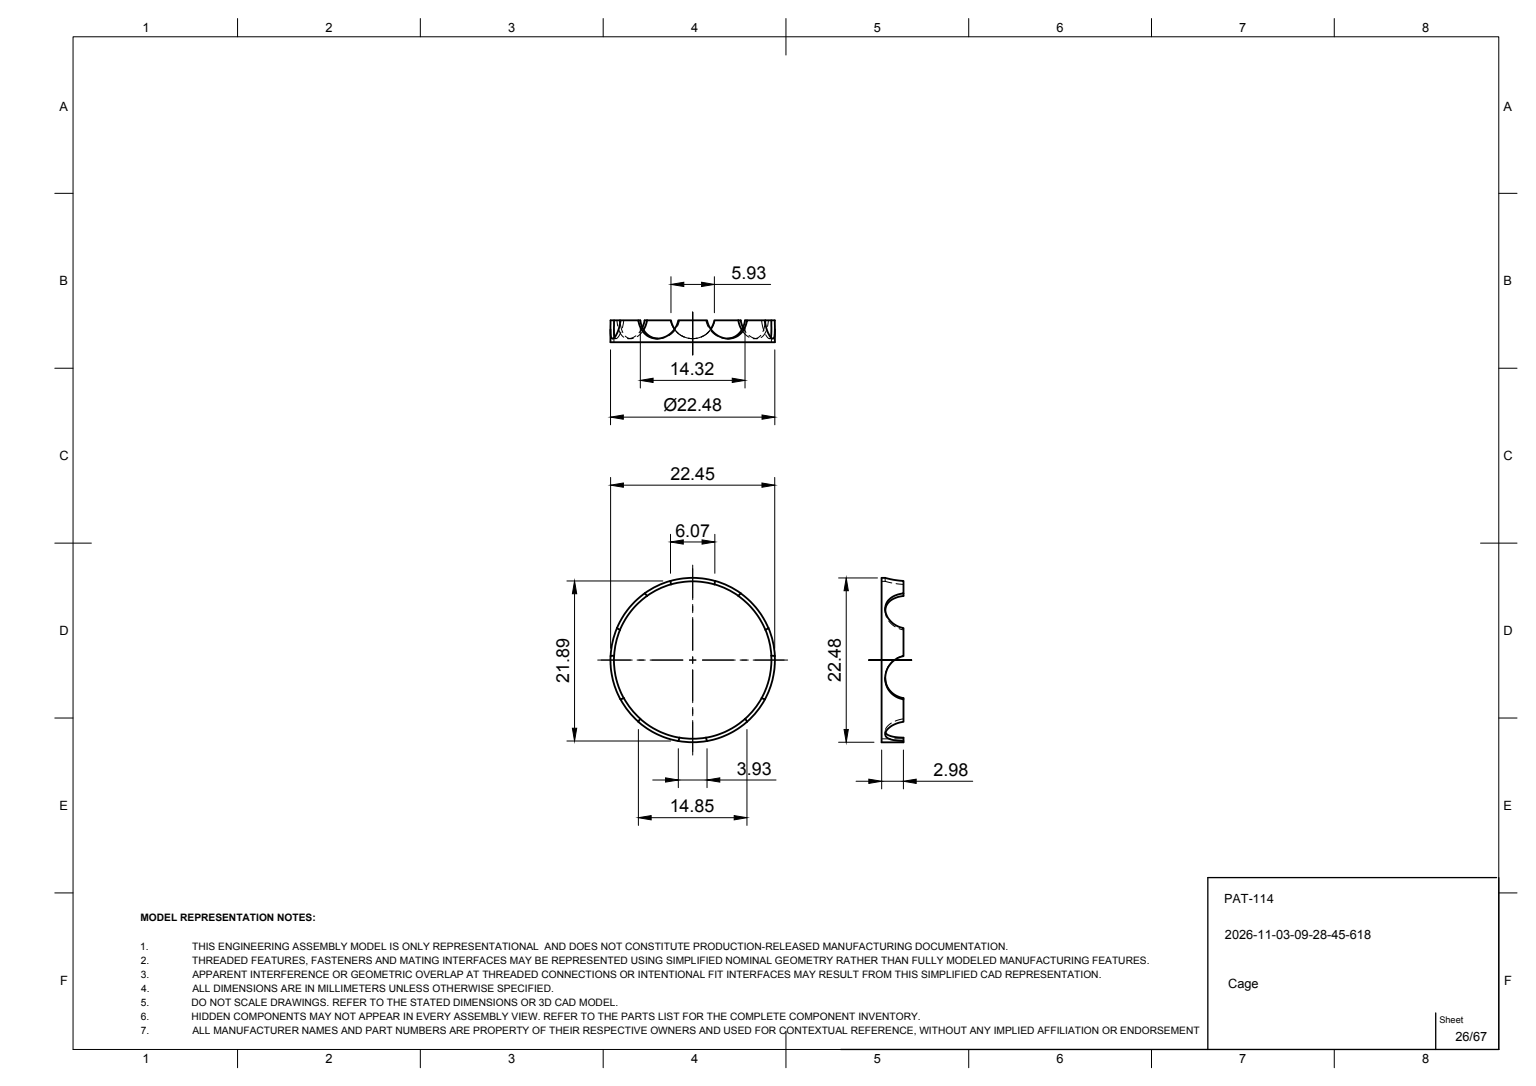
ISO-10303-21;
HEADER;
/* Generated by software containing ST-Developer
 * from STEP Tools, Inc. (www.steptools.com) 
 */

FILE_DESCRIPTION(
/* description */ ('Two-stage gear reducer in split housing'),
/* implementation_level */ '2;1');

FILE_NAME(
/* name */ 'Cage.step',
/* time_stamp */ '2026-10-28T03:22:31-07:00',
/* author */ (''),
/* organization */ (''),
/* preprocessor_version */ 'ST-DEVELOPER v20.2',
/* originating_system */ 'Autodesk Translation Framework v15.17.0.0',
/* authorisation */ '');

FILE_SCHEMA (('AUTOMOTIVE_DESIGN { 1 0 10303 214 3 1 1 }'));
ENDSEC;

DATA;
#10=MECHANICAL_DESIGN_GEOMETRIC_PRESENTATION_REPRESENTATION('',(#1260),#73366);
#931=B_SPLINE_CURVE_WITH_KNOTS('',3,(#24284,#24285,#24286,#24287,#24288,
#24289,#24290,#24291,#24292,#24293,#24294,#24295,#24296,#24297,#24298,#24299,
#24300,#24301,#24302,#24303,#24304,#24305),.UNSPECIFIED.,.F.,.F.,(4,2,2,
2,2,2,2,2,2,2,4),(0.0591825211272536,0.157966726598481,0.236950089897721,
0.315933453196962,0.391576304923761,0.46721915665056,0.54286200837736,0.618504860104159,
0.697488223403399,0.77647158670264,0.875255792173867),.UNSPECIFIED.);
#932=B_SPLINE_CURVE_WITH_KNOTS('',3,(#24309,#24310,#24311,#24312,#24313,
#24314,#24315,#24316,#24317,#24318,#24319,#24320,#24321,#24322,#24323,#24324,
#24325,#24326,#24327,#24328,#24329,#24330),.UNSPECIFIED.,.F.,.F.,(4,2,2,
2,2,2,2,2,2,2,4),(0.0581119756758434,0.106553146291161,0.213106292582322,
0.30849933801665,0.386091982889075,0.4636846277615,0.541277272633925,0.61886991750635,
0.714262962940678,0.820816109231839,0.869257279847157),.UNSPECIFIED.);
#933=B_SPLINE_CURVE_WITH_KNOTS('',3,(#24336,#24337,#24338,#24339,#24340,
#24341,#24342,#24343,#24344,#24345,#24346,#24347,#24348,#24349,#24350,#24351,
#24352,#24353,#24354,#24355,#24356,#24357),.UNSPECIFIED.,.F.,.F.,(4,2,2,
2,2,2,2,2,2,2,4),(0.0581119756758434,0.106553146291161,0.213106292582322,
0.30849933801665,0.386091982889075,0.4636846277615,0.541277272633925,0.61886991750635,
0.714262962940679,0.820816109231839,0.869257279847157),.UNSPECIFIED.);
#934=B_SPLINE_CURVE_WITH_KNOTS('',3,(#24361,#24362,#24363,#24364,#24365,
#24366,#24367,#24368,#24369,#24370,#24371,#24372,#24373,#24374,#24375,#24376,
#24377,#24378,#24379,#24380,#24381,#24382),.UNSPECIFIED.,.F.,.F.,(4,2,2,
2,2,2,2,2,2,2,4),(0.0581119756758433,0.106553146291161,0.213106292582322,
0.308499338016649,0.386091982889075,0.4636846277615,0.541277272633925,0.61886991750635,
0.714262962940678,0.820816109231839,0.869257279847157),.UNSPECIFIED.);
#935=B_SPLINE_CURVE_WITH_KNOTS('',3,(#24391,#24392,#24393,#24394,#24395,
#24396,#24397,#24398,#24399,#24400,#24401,#24402,#24403,#24404,#24405,#24406,
#24407,#24408,#24409,#24410,#24411,#24412),.UNSPECIFIED.,.F.,.F.,(4,2,2,
2,2,2,2,2,2,2,4),(0.0581119756758433,0.106553146291161,0.213106292582322,
0.30849933801665,0.386091982889075,0.4636846277615,0.541277272633925,0.61886991750635,
0.714262962940678,0.820816109231839,0.869257279847157),.UNSPECIFIED.);
#936=B_SPLINE_CURVE_WITH_KNOTS('',3,(#24416,#24417,#24418,#24419,#24420,
#24421,#24422,#24423,#24424,#24425,#24426,#24427,#24428,#24429,#24430,#24431,
#24432,#24433,#24434,#24435,#24436,#24437),.UNSPECIFIED.,.F.,.F.,(4,2,2,
2,2,2,2,2,2,2,4),(0.0581119756758434,0.106553146291161,0.213106292582322,
0.30849933801665,0.386091982889075,0.4636846277615,0.541277272633925,0.61886991750635,
0.714262962940678,0.820816109231839,0.869257279847157),.UNSPECIFIED.);
#937=B_SPLINE_CURVE_WITH_KNOTS('',3,(#24441,#24442,#24443,#24444,#24445,
#24446,#24447,#24448,#24449,#24450,#24451,#24452,#24453,#24454,#24455,#24456,
#24457,#24458,#24459,#24460,#24461,#24462),.UNSPECIFIED.,.F.,.F.,(4,2,2,
2,2,2,2,2,2,2,4),(0.0581119756758434,0.106553146291161,0.213106292582322,
0.30849933801665,0.386091982889075,0.4636846277615,0.541277272633925,0.61886991750635,
0.714262962940678,0.820816109231839,0.869257279847157),.UNSPECIFIED.);
#938=B_SPLINE_CURVE_WITH_KNOTS('',3,(#24466,#24467,#24468,#24469,#24470,
#24471,#24472,#24473,#24474,#24475,#24476,#24477,#24478,#24479,#24480,#24481,
#24482,#24483,#24484,#24485,#24486,#24487),.UNSPECIFIED.,.F.,.F.,(4,2,2,
2,2,2,2,2,2,2,4),(0.0581119756758433,0.106553146291161,0.213106292582322,
0.30849933801665,0.386091982889075,0.4636846277615,0.541277272633925,0.61886991750635,
0.714262962940678,0.820816109231839,0.869257279847157),.UNSPECIFIED.);
#939=B_SPLINE_CURVE_WITH_KNOTS('',3,(#24495,#24496,#24497,#24498,#24499,
#24500,#24501,#24502,#24503,#24504,#24505,#24506,#24507,#24508,#24509,#24510,
#24511,#24512,#24513,#24514,#24515,#24516),.UNSPECIFIED.,.F.,.F.,(4,2,2,
2,2,2,2,2,2,2,4),(0.0591825211272536,0.157966726598481,0.236950089897721,
0.315933453196962,0.391576304923761,0.467219156650561,0.54286200837736,
0.618504860104159,0.697488223403399,0.77647158670264,0.875255792173867),
 .UNSPECIFIED.);
#940=B_SPLINE_CURVE_WITH_KNOTS('',3,(#24524,#24525,#24526,#24527,#24528,
#24529,#24530,#24531,#24532,#24533,#24534,#24535,#24536,#24537,#24538,#24539,
#24540,#24541,#24542,#24543,#24544,#24545),.UNSPECIFIED.,.F.,.F.,(4,2,2,
2,2,2,2,2,2,2,4),(0.0591825211272536,0.157966726598481,0.236950089897722,
0.315933453196962,0.391576304923761,0.467219156650561,0.54286200837736,
0.618504860104159,0.697488223403399,0.77647158670264,0.875255792173867),
 .UNSPECIFIED.);
#941=B_SPLINE_CURVE_WITH_KNOTS('',3,(#24555,#24556,#24557,#24558,#24559,
#24560,#24561,#24562,#24563,#24564,#24565,#24566,#24567,#24568,#24569,#24570,
#24571,#24572,#24573,#24574,#24575,#24576),.UNSPECIFIED.,.F.,.F.,(4,2,2,
2,2,2,2,2,2,2,4),(0.0591825211272536,0.157966726598481,0.236950089897721,
0.315933453196962,0.391576304923761,0.46721915665056,0.54286200837736,0.618504860104159,
0.697488223403399,0.77647158670264,0.875255792173867),.UNSPECIFIED.);
#942=B_SPLINE_CURVE_WITH_KNOTS('',3,(#24584,#24585,#24586,#24587,#24588,
#24589,#24590,#24591,#24592,#24593,#24594,#24595,#24596,#24597,#24598,#24599,
#24600,#24601,#24602,#24603,#24604,#24605),.UNSPECIFIED.,.F.,.F.,(4,2,2,
2,2,2,2,2,2,2,4),(0.0591825211272536,0.157966726598481,0.236950089897721,
0.315933453196962,0.391576304923761,0.46721915665056,0.542862008377359,
0.618504860104159,0.697488223403399,0.776471586702639,0.875255792173867),
 .UNSPECIFIED.);
#943=B_SPLINE_CURVE_WITH_KNOTS('',3,(#24613,#24614,#24615,#24616,#24617,
#24618,#24619,#24620,#24621,#24622,#24623,#24624,#24625,#24626,#24627,#24628,
#24629,#24630,#24631,#24632,#24633,#24634),.UNSPECIFIED.,.F.,.F.,(4,2,2,
2,2,2,2,2,2,2,4),(0.0591825211272536,0.157966726598481,0.236950089897721,
0.315933453196962,0.391576304923761,0.46721915665056,0.54286200837736,0.618504860104159,
0.697488223403399,0.77647158670264,0.875255792173867),.UNSPECIFIED.);
#944=B_SPLINE_CURVE_WITH_KNOTS('',3,(#24643,#24644,#24645,#24646,#24647,
#24648,#24649,#24650,#24651,#24652,#24653,#24654,#24655,#24656,#24657,#24658,
#24659,#24660,#24661,#24662,#24663,#24664),.UNSPECIFIED.,.F.,.F.,(4,2,2,
2,2,2,2,2,2,2,4),(0.0591825211272536,0.157966726598481,0.236950089897721,
0.315933453196962,0.391576304923761,0.46721915665056,0.542862008377359,
0.618504860104159,0.697488223403399,0.776471586702639,0.875255792173867),
 .UNSPECIFIED.);
#1074=SPHERICAL_SURFACE('',#17473,0.309556);
#1075=SPHERICAL_SURFACE('',#17489,0.309556);
#1076=SPHERICAL_SURFACE('',#17494,0.309556);
#1077=SPHERICAL_SURFACE('',#17500,0.309556);
#1078=SPHERICAL_SURFACE('',#17505,0.309556);
#1079=SPHERICAL_SURFACE('',#17510,0.309556);
#1080=SPHERICAL_SURFACE('',#17518,0.309556);
#1142=SHAPE_REPRESENTATION_RELATIONSHIP('SRR','None',#73630,#1198);
#1198=ADVANCED_BREP_SHAPE_REPRESENTATION('',(#1330),#73326);
#1260=STYLED_ITEM('',(#73988),#1330);
#1330=MANIFOLD_SOLID_BREP('Continuous crown cage',#16149);
#1523=FACE_BOUND('',#3401,.T.);
#1759=PLANE('',#17486);
#1760=PLANE('',#17491);
#1761=PLANE('',#17496);
#1762=PLANE('',#17502);
#1763=PLANE('',#17507);
#1764=PLANE('',#17516);
#1765=PLANE('',#17520);
#1766=PLANE('',#17521);
#2323=FACE_OUTER_BOUND('',#3385,.T.);
#2324=FACE_OUTER_BOUND('',#3386,.T.);
#2325=FACE_OUTER_BOUND('',#3387,.T.);
#2326=FACE_OUTER_BOUND('',#3388,.T.);
#2327=FACE_OUTER_BOUND('',#3389,.T.);
#2328=FACE_OUTER_BOUND('',#3390,.T.);
#2329=FACE_OUTER_BOUND('',#3391,.T.);
#2330=FACE_OUTER_BOUND('',#3392,.T.);
#2331=FACE_OUTER_BOUND('',#3393,.T.);
#2332=FACE_OUTER_BOUND('',#3394,.T.);
#2333=FACE_OUTER_BOUND('',#3395,.T.);
#2334=FACE_OUTER_BOUND('',#3396,.T.);
#2335=FACE_OUTER_BOUND('',#3397,.T.);
#2336=FACE_OUTER_BOUND('',#3398,.T.);
#2337=FACE_OUTER_BOUND('',#3399,.T.);
#2338=FACE_OUTER_BOUND('',#3400,.T.);
#2339=FACE_OUTER_BOUND('',#3402,.T.);
#3385=EDGE_LOOP('',(#11893,#11894,#11895,#11896));
#3386=EDGE_LOOP('',(#11897,#11898,#11899,#11900,#11901,#11902,#11903,#11904,
#11905,#11906,#11907,#11908,#11909,#11910,#11911,#11912,#11913,#11914));
#3387=EDGE_LOOP('',(#11915,#11916,#11917,#11918));
#3388=EDGE_LOOP('',(#11919,#11920,#11921,#11922));
#3389=EDGE_LOOP('',(#11923,#11924,#11925,#11926));
#3390=EDGE_LOOP('',(#11927,#11928,#11929,#11930));
#3391=EDGE_LOOP('',(#11931,#11932,#11933,#11934,#11935,#11936));
#3392=EDGE_LOOP('',(#11937,#11938,#11939,#11940));
#3393=EDGE_LOOP('',(#11941,#11942,#11943,#11944));
#3394=EDGE_LOOP('',(#11945,#11946,#11947,#11948));
#3395=EDGE_LOOP('',(#11949,#11950,#11951,#11952));
#3396=EDGE_LOOP('',(#11953,#11954,#11955,#11956));
#3397=EDGE_LOOP('',(#11957,#11958,#11959,#11960,#11961,#11962,#11963,#11964,
#11965,#11966,#11967,#11968,#11969,#11970,#11971,#11972,#11973,#11974));
#3398=EDGE_LOOP('',(#11975,#11976,#11977,#11978));
#3399=EDGE_LOOP('',(#11979,#11980,#11981,#11982));
#3400=EDGE_LOOP('',(#11983));
#3401=EDGE_LOOP('',(#11984));
#3402=EDGE_LOOP('',(#11985,#11986,#11987,#11988));
#4433=LINE('',#24386,#5457);
#4434=LINE('',#24639,#5458);
#5457=VECTOR('',#20171,1.123812);
#5458=VECTOR('',#20240,1.076188);
#6420=CIRCLE('',#17474,0.303778037777585);
#6421=CIRCLE('',#17475,0.303778037777585);
#6422=CIRCLE('',#17477,1.123812);
#6423=CIRCLE('',#17478,1.123812);
#6424=CIRCLE('',#17479,1.123812);
#6425=CIRCLE('',#17480,1.123812);
#6426=CIRCLE('',#17481,1.123812);
#6427=CIRCLE('',#17482,1.123812);
#6428=CIRCLE('',#17483,1.123812);
#6429=CIRCLE('',#17484,1.123812);
#6430=CIRCLE('',#17485,1.123812);
#6431=CIRCLE('',#17487,1.076188);
#6432=CIRCLE('',#17488,0.303778037777585);
#6433=CIRCLE('',#17490,0.303778037777585);
#6434=CIRCLE('',#17492,1.076188);
#6435=CIRCLE('',#17493,0.303778037777585);
#6436=CIRCLE('',#17495,0.303778037777585);
#6437=CIRCLE('',#17497,1.076188);
#6438=CIRCLE('',#17498,1.076188);
#6439=CIRCLE('',#17499,0.303778037777585);
#6440=CIRCLE('',#17501,0.303778037777585);
#6441=CIRCLE('',#17503,1.076188);
#6442=CIRCLE('',#17504,0.303778037777585);
#6443=CIRCLE('',#17506,0.303778037777585);
#6444=CIRCLE('',#17508,1.076188);
#6445=CIRCLE('',#17509,0.303778037777585);
#6446=CIRCLE('',#17511,0.303778037777585);
#6447=CIRCLE('',#17513,1.076188);
#6448=CIRCLE('',#17514,1.076188);
#6449=CIRCLE('',#17515,1.076188);
#6450=CIRCLE('',#17517,0.303778037777585);
#6451=CIRCLE('',#17519,0.303778037777585);
#7293=VERTEX_POINT('',#24282);
#7294=VERTEX_POINT('',#24283);
#7295=VERTEX_POINT('',#24306);
#7296=VERTEX_POINT('',#24308);
#7297=VERTEX_POINT('',#24333);
#7298=VERTEX_POINT('',#24335);
#7299=VERTEX_POINT('',#24358);
#7300=VERTEX_POINT('',#24360);
#7301=VERTEX_POINT('',#24383);
#7302=VERTEX_POINT('',#24385);
#7303=VERTEX_POINT('',#24388);
#7304=VERTEX_POINT('',#24390);
#7305=VERTEX_POINT('',#24413);
#7306=VERTEX_POINT('',#24415);
#7307=VERTEX_POINT('',#24438);
#7308=VERTEX_POINT('',#24440);
#7309=VERTEX_POINT('',#24463);
#7310=VERTEX_POINT('',#24465);
#7311=VERTEX_POINT('',#24490);
#7312=VERTEX_POINT('',#24494);
#7313=VERTEX_POINT('',#24519);
#7314=VERTEX_POINT('',#24523);
#7315=VERTEX_POINT('',#24548);
#7316=VERTEX_POINT('',#24550);
#7317=VERTEX_POINT('',#24554);
#7318=VERTEX_POINT('',#24579);
#7319=VERTEX_POINT('',#24583);
#7320=VERTEX_POINT('',#24608);
#7321=VERTEX_POINT('',#24612);
#7322=VERTEX_POINT('',#24637);
#7323=VERTEX_POINT('',#24640);
#7324=VERTEX_POINT('',#24642);
#9000=EDGE_CURVE('',#7293,#7294,#931,.T.);
#9001=EDGE_CURVE('',#7295,#7293,#6420,.T.);
#9002=EDGE_CURVE('',#7296,#7295,#932,.T.);
#9003=EDGE_CURVE('',#7294,#7296,#6421,.T.);
#9004=EDGE_CURVE('',#7297,#7295,#6422,.T.);
#9005=EDGE_CURVE('',#7297,#7298,#933,.T.);
#9006=EDGE_CURVE('',#7299,#7298,#6423,.T.);
#9007=EDGE_CURVE('',#7299,#7300,#934,.T.);
#9008=EDGE_CURVE('',#7301,#7300,#6424,.T.);
#9009=EDGE_CURVE('',#7301,#7302,#4433,.T.);
#9010=EDGE_CURVE('',#7302,#7302,#6425,.T.);
#9011=EDGE_CURVE('',#7303,#7301,#6426,.T.);
#9012=EDGE_CURVE('',#7303,#7304,#935,.T.);
#9013=EDGE_CURVE('',#7305,#7304,#6427,.T.);
#9014=EDGE_CURVE('',#7305,#7306,#936,.T.);
#9015=EDGE_CURVE('',#7307,#7306,#6428,.T.);
#9016=EDGE_CURVE('',#7307,#7308,#937,.T.);
#9017=EDGE_CURVE('',#7309,#7308,#6429,.T.);
#9018=EDGE_CURVE('',#7309,#7310,#938,.T.);
#9019=EDGE_CURVE('',#7296,#7310,#6430,.T.);
#9020=EDGE_CURVE('',#7293,#7311,#6431,.T.);
#9021=EDGE_CURVE('',#7311,#7297,#6432,.T.);
#9022=EDGE_CURVE('',#7312,#7311,#939,.T.);
#9023=EDGE_CURVE('',#7298,#7312,#6433,.T.);
#9024=EDGE_CURVE('',#7312,#7313,#6434,.T.);
#9025=EDGE_CURVE('',#7313,#7299,#6435,.T.);
#9026=EDGE_CURVE('',#7314,#7313,#940,.T.);
#9027=EDGE_CURVE('',#7300,#7314,#6436,.T.);
#9028=EDGE_CURVE('',#7314,#7315,#6437,.T.);
#9029=EDGE_CURVE('',#7315,#7316,#6438,.T.);
#9030=EDGE_CURVE('',#7316,#7303,#6439,.T.);
#9031=EDGE_CURVE('',#7317,#7316,#941,.T.);
#9032=EDGE_CURVE('',#7304,#7317,#6440,.T.);
#9033=EDGE_CURVE('',#7317,#7318,#6441,.T.);
#9034=EDGE_CURVE('',#7318,#7305,#6442,.T.);
#9035=EDGE_CURVE('',#7319,#7318,#942,.T.);
#9036=EDGE_CURVE('',#7306,#7319,#6443,.T.);
#9037=EDGE_CURVE('',#7319,#7320,#6444,.T.);
#9038=EDGE_CURVE('',#7320,#7307,#6445,.T.);
#9039=EDGE_CURVE('',#7321,#7320,#943,.T.);
#9040=EDGE_CURVE('',#7308,#7321,#6446,.T.);
#9041=EDGE_CURVE('',#7322,#7322,#6447,.T.);
#9042=EDGE_CURVE('',#7322,#7315,#4434,.T.);
#9043=EDGE_CURVE('',#7323,#7294,#6448,.T.);
#9044=EDGE_CURVE('',#7323,#7324,#944,.T.);
#9045=EDGE_CURVE('',#7321,#7324,#6449,.T.);
#9046=EDGE_CURVE('',#7310,#7323,#6450,.T.);
#9047=EDGE_CURVE('',#7324,#7309,#6451,.T.);
#11893=ORIENTED_EDGE('',*,*,#9000,.F.);
#11894=ORIENTED_EDGE('',*,*,#9001,.F.);
#11895=ORIENTED_EDGE('',*,*,#9002,.F.);
#11896=ORIENTED_EDGE('',*,*,#9003,.F.);
#11897=ORIENTED_EDGE('',*,*,#9002,.T.);
#11898=ORIENTED_EDGE('',*,*,#9004,.F.);
#11899=ORIENTED_EDGE('',*,*,#9005,.T.);
#11900=ORIENTED_EDGE('',*,*,#9006,.F.);
#11901=ORIENTED_EDGE('',*,*,#9007,.T.);
#11902=ORIENTED_EDGE('',*,*,#9008,.F.);
#11903=ORIENTED_EDGE('',*,*,#9009,.T.);
#11904=ORIENTED_EDGE('',*,*,#9010,.F.);
#11905=ORIENTED_EDGE('',*,*,#9009,.F.);
#11906=ORIENTED_EDGE('',*,*,#9011,.F.);
#11907=ORIENTED_EDGE('',*,*,#9012,.T.);
#11908=ORIENTED_EDGE('',*,*,#9013,.F.);
#11909=ORIENTED_EDGE('',*,*,#9014,.T.);
#11910=ORIENTED_EDGE('',*,*,#9015,.F.);
#11911=ORIENTED_EDGE('',*,*,#9016,.T.);
#11912=ORIENTED_EDGE('',*,*,#9017,.F.);
#11913=ORIENTED_EDGE('',*,*,#9018,.T.);
#11914=ORIENTED_EDGE('',*,*,#9019,.F.);
#11915=ORIENTED_EDGE('',*,*,#9001,.T.);
#11916=ORIENTED_EDGE('',*,*,#9020,.T.);
#11917=ORIENTED_EDGE('',*,*,#9021,.T.);
#11918=ORIENTED_EDGE('',*,*,#9004,.T.);
#11919=ORIENTED_EDGE('',*,*,#9022,.F.);
#11920=ORIENTED_EDGE('',*,*,#9023,.F.);
#11921=ORIENTED_EDGE('',*,*,#9005,.F.);
#11922=ORIENTED_EDGE('',*,*,#9021,.F.);
#11923=ORIENTED_EDGE('',*,*,#9023,.T.);
#11924=ORIENTED_EDGE('',*,*,#9024,.T.);
#11925=ORIENTED_EDGE('',*,*,#9025,.T.);
#11926=ORIENTED_EDGE('',*,*,#9006,.T.);
#11927=ORIENTED_EDGE('',*,*,#9026,.F.);
#11928=ORIENTED_EDGE('',*,*,#9027,.F.);
#11929=ORIENTED_EDGE('',*,*,#9007,.F.);
#11930=ORIENTED_EDGE('',*,*,#9025,.F.);
#11931=ORIENTED_EDGE('',*,*,#9027,.T.);
#11932=ORIENTED_EDGE('',*,*,#9028,.T.);
#11933=ORIENTED_EDGE('',*,*,#9029,.T.);
#11934=ORIENTED_EDGE('',*,*,#9030,.T.);
#11935=ORIENTED_EDGE('',*,*,#9011,.T.);
#11936=ORIENTED_EDGE('',*,*,#9008,.T.);
#11937=ORIENTED_EDGE('',*,*,#9031,.F.);
#11938=ORIENTED_EDGE('',*,*,#9032,.F.);
#11939=ORIENTED_EDGE('',*,*,#9012,.F.);
#11940=ORIENTED_EDGE('',*,*,#9030,.F.);
#11941=ORIENTED_EDGE('',*,*,#9032,.T.);
#11942=ORIENTED_EDGE('',*,*,#9033,.T.);
#11943=ORIENTED_EDGE('',*,*,#9034,.T.);
#11944=ORIENTED_EDGE('',*,*,#9013,.T.);
#11945=ORIENTED_EDGE('',*,*,#9035,.F.);
#11946=ORIENTED_EDGE('',*,*,#9036,.F.);
#11947=ORIENTED_EDGE('',*,*,#9014,.F.);
#11948=ORIENTED_EDGE('',*,*,#9034,.F.);
#11949=ORIENTED_EDGE('',*,*,#9036,.T.);
#11950=ORIENTED_EDGE('',*,*,#9037,.T.);
#11951=ORIENTED_EDGE('',*,*,#9038,.T.);
#11952=ORIENTED_EDGE('',*,*,#9015,.T.);
#11953=ORIENTED_EDGE('',*,*,#9016,.F.);
#11954=ORIENTED_EDGE('',*,*,#9038,.F.);
#11955=ORIENTED_EDGE('',*,*,#9039,.F.);
#11956=ORIENTED_EDGE('',*,*,#9040,.F.);
#11957=ORIENTED_EDGE('',*,*,#9041,.F.);
#11958=ORIENTED_EDGE('',*,*,#9042,.T.);
#11959=ORIENTED_EDGE('',*,*,#9028,.F.);
#11960=ORIENTED_EDGE('',*,*,#9026,.T.);
#11961=ORIENTED_EDGE('',*,*,#9024,.F.);
#11962=ORIENTED_EDGE('',*,*,#9022,.T.);
#11963=ORIENTED_EDGE('',*,*,#9020,.F.);
#11964=ORIENTED_EDGE('',*,*,#9000,.T.);
#11965=ORIENTED_EDGE('',*,*,#9043,.F.);
#11966=ORIENTED_EDGE('',*,*,#9044,.T.);
#11967=ORIENTED_EDGE('',*,*,#9045,.F.);
#11968=ORIENTED_EDGE('',*,*,#9039,.T.);
#11969=ORIENTED_EDGE('',*,*,#9037,.F.);
#11970=ORIENTED_EDGE('',*,*,#9035,.T.);
#11971=ORIENTED_EDGE('',*,*,#9033,.F.);
#11972=ORIENTED_EDGE('',*,*,#9031,.T.);
#11973=ORIENTED_EDGE('',*,*,#9029,.F.);
#11974=ORIENTED_EDGE('',*,*,#9042,.F.);
#11975=ORIENTED_EDGE('',*,*,#9003,.T.);
#11976=ORIENTED_EDGE('',*,*,#9019,.T.);
#11977=ORIENTED_EDGE('',*,*,#9046,.T.);
#11978=ORIENTED_EDGE('',*,*,#9043,.T.);
#11979=ORIENTED_EDGE('',*,*,#9018,.F.);
#11980=ORIENTED_EDGE('',*,*,#9047,.F.);
#11981=ORIENTED_EDGE('',*,*,#9044,.F.);
#11982=ORIENTED_EDGE('',*,*,#9046,.F.);
#11983=ORIENTED_EDGE('',*,*,#9010,.T.);
#11984=ORIENTED_EDGE('',*,*,#9041,.T.);
#11985=ORIENTED_EDGE('',*,*,#9040,.T.);
#11986=ORIENTED_EDGE('',*,*,#9045,.T.);
#11987=ORIENTED_EDGE('',*,*,#9047,.T.);
#11988=ORIENTED_EDGE('',*,*,#9017,.T.);
#15055=CYLINDRICAL_SURFACE('',#17476,1.123812);
#15056=CYLINDRICAL_SURFACE('',#17512,1.076188);
#15530=ADVANCED_FACE('',(#2323),#1074,.F.);
#15531=ADVANCED_FACE('',(#2324),#15055,.T.);
#15532=ADVANCED_FACE('',(#2325),#1759,.T.);
#15533=ADVANCED_FACE('',(#2326),#1075,.F.);
#15534=ADVANCED_FACE('',(#2327),#1760,.T.);
#15535=ADVANCED_FACE('',(#2328),#1076,.F.);
#15536=ADVANCED_FACE('',(#2329),#1761,.T.);
#15537=ADVANCED_FACE('',(#2330),#1077,.F.);
#15538=ADVANCED_FACE('',(#2331),#1762,.T.);
#15539=ADVANCED_FACE('',(#2332),#1078,.F.);
#15540=ADVANCED_FACE('',(#2333),#1763,.T.);
#15541=ADVANCED_FACE('',(#2334),#1079,.F.);
#15542=ADVANCED_FACE('',(#2335),#15056,.F.);
#15543=ADVANCED_FACE('',(#2336),#1764,.T.);
#15544=ADVANCED_FACE('',(#2337),#1080,.F.);
#15545=ADVANCED_FACE('',(#2338,#1523),#1765,.T.);
#15546=ADVANCED_FACE('',(#2339),#1766,.T.);
#16149=CLOSED_SHELL('',(#15530,#15531,#15532,#15533,#15534,#15535,#15536,
#15537,#15538,#15539,#15540,#15541,#15542,#15543,#15544,#15545,#15546));
#17472=AXIS2_PLACEMENT_3D('',#24280,#20155,#20156);
#17473=AXIS2_PLACEMENT_3D('',#24281,#20157,#20158);
#17474=AXIS2_PLACEMENT_3D('',#24307,#20159,#20160);
#17475=AXIS2_PLACEMENT_3D('',#24331,#20161,#20162);
#17476=AXIS2_PLACEMENT_3D('',#24332,#20163,#20164);
#17477=AXIS2_PLACEMENT_3D('',#24334,#20165,#20166);
#17478=AXIS2_PLACEMENT_3D('',#24359,#20167,#20168);
#17479=AXIS2_PLACEMENT_3D('',#24384,#20169,#20170);
#17480=AXIS2_PLACEMENT_3D('',#24387,#20172,#20173);
#17481=AXIS2_PLACEMENT_3D('',#24389,#20174,#20175);
#17482=AXIS2_PLACEMENT_3D('',#24414,#20176,#20177);
#17483=AXIS2_PLACEMENT_3D('',#24439,#20178,#20179);
#17484=AXIS2_PLACEMENT_3D('',#24464,#20180,#20181);
#17485=AXIS2_PLACEMENT_3D('',#24488,#20182,#20183);
#17486=AXIS2_PLACEMENT_3D('',#24489,#20184,#20185);
#17487=AXIS2_PLACEMENT_3D('',#24491,#20186,#20187);
#17488=AXIS2_PLACEMENT_3D('',#24492,#20188,#20189);
#17489=AXIS2_PLACEMENT_3D('',#24493,#20190,#20191);
#17490=AXIS2_PLACEMENT_3D('',#24517,#20192,#20193);
#17491=AXIS2_PLACEMENT_3D('',#24518,#20194,#20195);
#17492=AXIS2_PLACEMENT_3D('',#24520,#20196,#20197);
#17493=AXIS2_PLACEMENT_3D('',#24521,#20198,#20199);
#17494=AXIS2_PLACEMENT_3D('',#24522,#20200,#20201);
#17495=AXIS2_PLACEMENT_3D('',#24546,#20202,#20203);
#17496=AXIS2_PLACEMENT_3D('',#24547,#20204,#20205);
#17497=AXIS2_PLACEMENT_3D('',#24549,#20206,#20207);
#17498=AXIS2_PLACEMENT_3D('',#24551,#20208,#20209);
#17499=AXIS2_PLACEMENT_3D('',#24552,#20210,#20211);
#17500=AXIS2_PLACEMENT_3D('',#24553,#20212,#20213);
#17501=AXIS2_PLACEMENT_3D('',#24577,#20214,#20215);
#17502=AXIS2_PLACEMENT_3D('',#24578,#20216,#20217);
#17503=AXIS2_PLACEMENT_3D('',#24580,#20218,#20219);
#17504=AXIS2_PLACEMENT_3D('',#24581,#20220,#20221);
#17505=AXIS2_PLACEMENT_3D('',#24582,#20222,#20223);
#17506=AXIS2_PLACEMENT_3D('',#24606,#20224,#20225);
#17507=AXIS2_PLACEMENT_3D('',#24607,#20226,#20227);
#17508=AXIS2_PLACEMENT_3D('',#24609,#20228,#20229);
#17509=AXIS2_PLACEMENT_3D('',#24610,#20230,#20231);
#17510=AXIS2_PLACEMENT_3D('',#24611,#20232,#20233);
#17511=AXIS2_PLACEMENT_3D('',#24635,#20234,#20235);
#17512=AXIS2_PLACEMENT_3D('',#24636,#20236,#20237);
#17513=AXIS2_PLACEMENT_3D('',#24638,#20238,#20239);
#17514=AXIS2_PLACEMENT_3D('',#24641,#20241,#20242);
#17515=AXIS2_PLACEMENT_3D('',#24665,#20243,#20244);
#17516=AXIS2_PLACEMENT_3D('',#24666,#20245,#20246);
#17517=AXIS2_PLACEMENT_3D('',#24667,#20247,#20248);
#17518=AXIS2_PLACEMENT_3D('',#24668,#20249,#20250);
#17519=AXIS2_PLACEMENT_3D('',#24669,#20251,#20252);
#17520=AXIS2_PLACEMENT_3D('',#24670,#20253,#20254);
#17521=AXIS2_PLACEMENT_3D('',#24671,#20255,#20256);
#20155=DIRECTION('axis',(0.,0.,1.));
#20156=DIRECTION('refdir',(1.,0.,0.));
#20157=DIRECTION('center_axis',(0.,0.,1.));
#20158=DIRECTION('ref_axis',(1.,0.,0.));
#20159=DIRECTION('center_axis',(0.,-1.,0.));
#20160=DIRECTION('ref_axis',(0.,0.,-1.));
#20161=DIRECTION('center_axis',(0.,-1.,0.));
#20162=DIRECTION('ref_axis',(0.,0.,-1.));
#20163=DIRECTION('center_axis',(0.,1.,0.));
#20164=DIRECTION('ref_axis',(1.,0.,0.));
#20165=DIRECTION('center_axis',(0.,1.,0.));
#20166=DIRECTION('ref_axis',(1.,0.,0.));
#20167=DIRECTION('center_axis',(0.,1.,0.));
#20168=DIRECTION('ref_axis',(1.,0.,0.));
#20169=DIRECTION('center_axis',(0.,1.,0.));
#20170=DIRECTION('ref_axis',(1.,0.,0.));
#20171=DIRECTION('',(0.,-1.,0.));
#20172=DIRECTION('center_axis',(0.,-1.,0.));
#20173=DIRECTION('ref_axis',(1.,0.,0.));
#20174=DIRECTION('center_axis',(0.,1.,0.));
#20175=DIRECTION('ref_axis',(1.,0.,0.));
#20176=DIRECTION('center_axis',(0.,1.,0.));
#20177=DIRECTION('ref_axis',(1.,0.,0.));
#20178=DIRECTION('center_axis',(0.,1.,0.));
#20179=DIRECTION('ref_axis',(1.,0.,0.));
#20180=DIRECTION('center_axis',(0.,1.,0.));
#20181=DIRECTION('ref_axis',(1.,0.,0.));
#20182=DIRECTION('center_axis',(0.,1.,0.));
#20183=DIRECTION('ref_axis',(1.,0.,0.));
#20184=DIRECTION('center_axis',(0.,1.,0.));
#20185=DIRECTION('ref_axis',(1.,0.,0.));
#20186=DIRECTION('center_axis',(0.,-1.,0.));
#20187=DIRECTION('ref_axis',(1.,0.,0.));
#20188=DIRECTION('center_axis',(0.,-1.,0.));
#20189=DIRECTION('ref_axis',(0.,0.,-1.));
#20190=DIRECTION('center_axis',(8.96625347776458E-17,0.,1.));
#20191=DIRECTION('ref_axis',(1.,0.,0.));
#20192=DIRECTION('center_axis',(0.,-1.,0.));
#20193=DIRECTION('ref_axis',(0.,0.,-1.));
#20194=DIRECTION('center_axis',(0.,1.,0.));
#20195=DIRECTION('ref_axis',(1.,0.,0.));
#20196=DIRECTION('center_axis',(0.,-1.,0.));
#20197=DIRECTION('ref_axis',(1.,0.,0.));
#20198=DIRECTION('center_axis',(0.,-1.,0.));
#20199=DIRECTION('ref_axis',(0.,0.,-1.));
#20200=DIRECTION('center_axis',(0.,0.,1.));
#20201=DIRECTION('ref_axis',(1.,0.,0.));
#20202=DIRECTION('center_axis',(0.,-1.,0.));
#20203=DIRECTION('ref_axis',(0.,0.,-1.));
#20204=DIRECTION('center_axis',(0.,1.,0.));
#20205=DIRECTION('ref_axis',(1.,0.,0.));
#20206=DIRECTION('center_axis',(0.,-1.,0.));
#20207=DIRECTION('ref_axis',(1.,0.,0.));
#20208=DIRECTION('center_axis',(0.,-1.,0.));
#20209=DIRECTION('ref_axis',(1.,0.,0.));
#20210=DIRECTION('center_axis',(0.,-1.,0.));
#20211=DIRECTION('ref_axis',(0.,0.,-1.));
#20212=DIRECTION('center_axis',(0.,0.,1.));
#20213=DIRECTION('ref_axis',(1.,0.,0.));
#20214=DIRECTION('center_axis',(0.,-1.,0.));
#20215=DIRECTION('ref_axis',(0.,0.,-1.));
#20216=DIRECTION('center_axis',(0.,1.,0.));
#20217=DIRECTION('ref_axis',(1.,0.,0.));
#20218=DIRECTION('center_axis',(0.,-1.,0.));
#20219=DIRECTION('ref_axis',(1.,0.,0.));
#20220=DIRECTION('center_axis',(0.,-1.,0.));
#20221=DIRECTION('ref_axis',(0.,0.,-1.));
#20222=DIRECTION('center_axis',(8.96625347776458E-17,0.,1.));
#20223=DIRECTION('ref_axis',(1.,0.,0.));
#20224=DIRECTION('center_axis',(0.,-1.,0.));
#20225=DIRECTION('ref_axis',(0.,0.,-1.));
#20226=DIRECTION('center_axis',(0.,1.,0.));
#20227=DIRECTION('ref_axis',(1.,0.,0.));
#20228=DIRECTION('center_axis',(0.,-1.,0.));
#20229=DIRECTION('ref_axis',(1.,0.,0.));
#20230=DIRECTION('center_axis',(0.,-1.,0.));
#20231=DIRECTION('ref_axis',(0.,0.,-1.));
#20232=DIRECTION('center_axis',(0.,0.,1.));
#20233=DIRECTION('ref_axis',(1.,0.,0.));
#20234=DIRECTION('center_axis',(0.,-1.,0.));
#20235=DIRECTION('ref_axis',(0.,0.,-1.));
#20236=DIRECTION('center_axis',(0.,1.,0.));
#20237=DIRECTION('ref_axis',(1.,0.,0.));
#20238=DIRECTION('center_axis',(0.,1.,0.));
#20239=DIRECTION('ref_axis',(1.,0.,0.));
#20240=DIRECTION('',(0.,1.,0.));
#20241=DIRECTION('center_axis',(0.,-1.,0.));
#20242=DIRECTION('ref_axis',(1.,0.,0.));
#20243=DIRECTION('center_axis',(0.,-1.,0.));
#20244=DIRECTION('ref_axis',(1.,0.,0.));
#20245=DIRECTION('center_axis',(0.,1.,0.));
#20246=DIRECTION('ref_axis',(1.,0.,0.));
#20247=DIRECTION('center_axis',(0.,-1.,0.));
#20248=DIRECTION('ref_axis',(0.,0.,-1.));
#20249=DIRECTION('center_axis',(0.,0.,1.));
#20250=DIRECTION('ref_axis',(1.,0.,0.));
#20251=DIRECTION('center_axis',(0.,-1.,0.));
#20252=DIRECTION('ref_axis',(0.,0.,-1.));
#20253=DIRECTION('center_axis',(0.,-1.,0.));
#20254=DIRECTION('ref_axis',(-1.,0.,0.));
#20255=DIRECTION('center_axis',(0.,1.,0.));
#20256=DIRECTION('ref_axis',(1.,0.,0.));
#24280=CARTESIAN_POINT('',(0.,0.,0.));
#24281=CARTESIAN_POINT('Origin',(0.685838782044607,0.,0.860014630714833));
#24282=CARTESIAN_POINT('',(0.413083465285518,-0.05953,0.993751811093549));
#24283=CARTESIAN_POINT('',(0.876916659919095,-0.05953,0.623857181492959));
#24284=CARTESIAN_POINT('Ctrl Pts',(0.413083465285518,-0.05953,0.993751811093549));
#24285=CARTESIAN_POINT('Ctrl Pts',(0.419070565453383,-0.0925528133349865,
0.991263089003441));
#24286=CARTESIAN_POINT('Ctrl Pts',(0.430199341854858,-0.124911173756694,
0.986608710139579));
#24287=CARTESIAN_POINT('Ctrl Pts',(0.457978755888596,-0.177924977804098,
0.973971221090534));
#24288=CARTESIAN_POINT('Ctrl Pts',(0.473077587363685,-0.199697230012983,
0.966820759530997));
#24289=CARTESIAN_POINT('Ctrl Pts',(0.507057380724533,-0.237895043532788,
0.949440676105255));
#24290=CARTESIAN_POINT('Ctrl Pts',(0.525933334162555,-0.254319232363049,
0.939198248544428));
#24291=CARTESIAN_POINT('Ctrl Pts',(0.564362943424238,-0.28018331644634,
0.916597376014514));
#24292=CARTESIAN_POINT('Ctrl Pts',(0.585840553788742,-0.29104845371857,
0.903141581680914));
#24293=CARTESIAN_POINT('Ctrl Pts',(0.629305439856167,-0.30527573347708,
0.873412008702649));
#24294=CARTESIAN_POINT('Ctrl Pts',(0.651278921914856,-0.308638795020976,
0.857118508332695));
#24295=CARTESIAN_POINT('Ctrl Pts',(0.690705563850638,-0.308638795020976,
0.825676810575914));
#24296=CARTESIAN_POINT('Ctrl Pts',(0.711480111898423,-0.30527573347708,
0.807879894508811));
#24297=CARTESIAN_POINT('Ctrl Pts',(0.750136149454208,-0.29104845371857,
0.772120216227122));
#24298=CARTESIAN_POINT('Ctrl Pts',(0.768033796848072,-0.28018331644634,
0.754175290318038));
#24299=CARTESIAN_POINT('Ctrl Pts',(0.798619410861634,-0.254319232363049,
0.721738358858166));
#24300=CARTESIAN_POINT('Ctrl Pts',(0.812805334167529,-0.237895043532788,
0.705614819529209));
#24301=CARTESIAN_POINT('Ctrl Pts',(0.837310877969633,-0.199697230012983,
0.676354402927683));
#24302=CARTESIAN_POINT('Ctrl Pts',(0.847641868610495,-0.177924977804098,
0.663225258065736));
#24303=CARTESIAN_POINT('Ctrl Pts',(0.866144010579847,-0.124911173756694,
0.638954437806245));
#24304=CARTESIAN_POINT('Ctrl Pts',(0.873158080166742,-0.0925528133349865,
0.62914037979579));
#24305=CARTESIAN_POINT('Ctrl Pts',(0.876916659919095,-0.05953,0.623857181492959));
#24306=CARTESIAN_POINT('',(0.437601487681057,-0.05953,1.03511272300331));
#24307=CARTESIAN_POINT('Origin',(0.685838782044607,-0.05953,0.860014630714833));
#24308=CARTESIAN_POINT('',(0.911784794170997,-0.05953,0.656964154625313));
#24309=CARTESIAN_POINT('Ctrl Pts',(0.911784794170998,-0.0595300000000001,
0.656964154625312));
#24310=CARTESIAN_POINT('Ctrl Pts',(0.909827729890942,-0.0762225747374255,
0.659680317203144));
#24311=CARTESIAN_POINT('Ctrl Pts',(0.907004864562642,-0.0928409665394228,
0.663576540841106));
#24312=CARTESIAN_POINT('Ctrl Pts',(0.895234408667242,-0.144299303100741,
0.679480524217551));
#24313=CARTESIAN_POINT('Ctrl Pts',(0.882797231409153,-0.177024326825049,
0.695831250979106));
#24314=CARTESIAN_POINT('Ctrl Pts',(0.854332839576145,-0.227269801620064,
0.73042219438957));
#24315=CARTESIAN_POINT('Ctrl Pts',(0.834863020612702,-0.251265615809407,
0.752807465209441));
#24316=CARTESIAN_POINT('Ctrl Pts',(0.800439809856111,-0.279889827963178,
0.789147407129766));
#24317=CARTESIAN_POINT('Ctrl Pts',(0.781998747691871,-0.290879136862659,
0.80756613568454));
#24318=CARTESIAN_POINT('Ctrl Pts',(0.742239891936898,-0.305251990234487,
0.844254137480382));
#24319=CARTESIAN_POINT('Ctrl Pts',(0.720906778729541,-0.308638795020976,
0.862505527716294));
#24320=CARTESIAN_POINT('Ctrl Pts',(0.680463863683392,-0.308638795020976,
0.894757676234429));
#24321=CARTESIAN_POINT('Ctrl Pts',(0.657923009631182,-0.305251990234488,
0.91149460735272));
#24322=CARTESIAN_POINT('Ctrl Pts',(0.613307674922609,-0.290879136862659,
0.942092777160053));
#24323=CARTESIAN_POINT('Ctrl Pts',(0.591247219971725,-0.279889827963178,
0.955972930713954));
#24324=CARTESIAN_POINT('Ctrl Pts',(0.548158511259202,-0.251265615809407,
0.981446681891443));
#24325=CARTESIAN_POINT('Ctrl Pts',(0.522002043615455,-0.227269801620063,
0.995447160474328));
#24326=CARTESIAN_POINT('Ctrl Pts',(0.481944444320713,-0.177024326825049,
1.01550068154148));
#24327=CARTESIAN_POINT('Ctrl Pts',(0.463236132117164,-0.14429930310074,
1.0239876538093));
#24328=CARTESIAN_POINT('Ctrl Pts',(0.445111721969657,-0.0928409665394226,
1.03192403056628));
#24329=CARTESIAN_POINT('Ctrl Pts',(0.440685038163619,-0.0762225747374254,
1.03380912944435));
#24330=CARTESIAN_POINT('Ctrl Pts',(0.437601487681056,-0.05953,1.03511272300331));
#24331=CARTESIAN_POINT('Origin',(0.685838782044607,-0.05953,0.860014630714833));
#24332=CARTESIAN_POINT('Origin',(0.,-0.208355,0.));
#24333=CARTESIAN_POINT('',(0.0548532617164168,-0.05953,1.12247250791415));
#24334=CARTESIAN_POINT('Origin',(0.,-0.05953,0.));
#24335=CARTESIAN_POINT('',(-0.536443649899848,-0.05953,0.987512846410683));
#24336=CARTESIAN_POINT('Ctrl Pts',(0.0548532617164173,-0.0595300000000001,
1.12247250791414));
#24337=CARTESIAN_POINT('Ctrl Pts',(0.05150947068137,-0.0762225747374254,
1.12263591311425));
#24338=CARTESIAN_POINT('Ctrl Pts',(0.0467032526342597,-0.0928409665394227,
1.12285816383385));
#24339=CARTESIAN_POINT('Ctrl Pts',(0.0269302585198975,-0.144299303100741,
1.12357162229597));
#24340=CARTESIAN_POINT('Ctrl Pts',(0.006392292392153,-0.177024326825049,
1.12404235695137));
#24341=CARTESIAN_POINT('Ctrl Pts',(-0.0383992541984087,-0.227269801620063,
1.12335509974011));
#24342=CARTESIAN_POINT('Ctrl Pts',(-0.0680399972366993,-0.251265615809407,
1.12208997038458));
#24343=CARTESIAN_POINT('Ctrl Pts',(-0.117914228755037,-0.279889827963178,
1.1178344036749));
#24344=CARTESIAN_POINT('Ctrl Pts',(-0.14381238480104,-0.290879136862659,
1.11490049012186));
#24345=CARTESIAN_POINT('Ctrl Pts',(-0.19728546073067,-0.305251990234488,
1.10669035995599));
#24346=CARTESIAN_POINT('Ctrl Pts',(-0.224855950742601,-0.308638795020976,
1.10139101611326));
#24347=CARTESIAN_POINT('Ctrl Pts',(-0.275287440920027,-0.308638795020976,
1.0898803575765));
#24348=CARTESIAN_POINT('Ctrl Pts',(-0.302426893214945,-0.305251990234488,
1.08269251410343));
#24349=CARTESIAN_POINT('Ctrl Pts',(-0.35416671187353,-0.290879136862659,
1.06688848765783));
#24350=CARTESIAN_POINT('Ctrl Pts',(-0.3787731215897,-0.279889827963178,
1.05829506364875));
#24351=CARTESIAN_POINT('Ctrl Pts',(-0.425554672694338,-0.251265615809407,
1.04048957871266));
#24352=CARTESIAN_POINT('Ctrl Pts',(-0.452808978448581,-0.227269801620063,
1.02876878445619));
#24353=CARTESIAN_POINT('Ctrl Pts',(-0.493462957200432,-0.177024326825049,
1.0099536580922));
#24354=CARTESIAN_POINT('Ctrl Pts',(-0.511762781179148,-0.14429930310074,
1.00061845128527));
#24355=CARTESIAN_POINT('Ctrl Pts',(-0.529268075276157,-0.0928409665394226,
0.991396466802468));
#24356=CARTESIAN_POINT('Ctrl Pts',(-0.533501897135713,-0.0762225747374254,
0.989110885965947));
#24357=CARTESIAN_POINT('Ctrl Pts',(-0.536443649899848,-0.0595300000000001,
0.987512846410683));
#24358=CARTESIAN_POINT('',(-0.843383895613249,-0.05953,0.742736168477219));
#24359=CARTESIAN_POINT('Origin',(0.,-0.05953,0.));
#24360=CARTESIAN_POINT('',(-1.10653577764992,-0.05953,0.196295654879792));
#24361=CARTESIAN_POINT('Ctrl Pts',(-0.843383895613249,-0.0595300000000001,
0.742736168477219));
#24362=CARTESIAN_POINT('Ctrl Pts',(-0.84559647055299,-0.0762225747374255,
0.740223768851062));
#24363=CARTESIAN_POINT('Ctrl Pts',(-0.848766861100456,-0.0928409665394227,
0.736604687327351));
#24364=CARTESIAN_POINT('Ctrl Pts',(-0.861652925570091,-0.144299303100741,
0.721590372101268));
#24365=CARTESIAN_POINT('Ctrl Pts',(-0.87482617317514,-0.177024326825049,
0.705826641853758));
#24366=CARTESIAN_POINT('Ctrl Pts',(-0.902215926359523,-0.227269801620063,
0.670378702718353));
#24367=CARTESIAN_POINT('Ctrl Pts',(-0.919707509403859,-0.251265615809407,
0.646415841396062));
#24368=CARTESIAN_POINT('Ctrl Pts',(-0.947476448101718,-0.279889827963178,
0.604769294586516));
#24369=CARTESIAN_POINT('Ctrl Pts',(-0.961329858300736,-0.290879136862659,
0.582692035672022));
#24370=CARTESIAN_POINT('Ctrl Pts',(-0.988250837578047,-0.305251990234488,
0.535766169015486));
#24371=CARTESIAN_POINT('Ctrl Pts',(-1.00129756308006,-0.308638795020976,
0.510906605094603));
#24372=CARTESIAN_POINT('Ctrl Pts',(-1.02374168767024,-0.308638795020976,
0.46430090015576));
#24373=CARTESIAN_POINT('Ctrl Pts',(-1.03504317708586,-0.305251990234488,
0.438600874831839));
#24374=CARTESIAN_POINT('Ctrl Pts',(-1.05494634094458,-0.290879136862659,
0.388295406390235));
#24375=CARTESIAN_POINT('Ctrl Pts',(-1.06356957703048,-0.279889827963178,
0.363699428370917));
#24376=CARTESIAN_POINT('Ctrl Pts',(-1.0788165083757,-0.251265615809407,
0.316022600643821));
#24377=CARTESIAN_POINT('Ctrl Pts',(-1.08664560412098,-0.227269801620063,
0.287406530683752));
#24378=CARTESIAN_POINT('Ctrl Pts',(-1.09728268713976,-0.177024326825049,
0.243890930799337));
#24379=CARTESIAN_POINT('Ctrl Pts',(-1.10139388218929,-0.144299303100741,
0.22376314604679));
#24380=CARTESIAN_POINT('Ctrl Pts',(-1.10509821673782,-0.0928409665394227,
0.204327142733961));
#24381=CARTESIAN_POINT('Ctrl Pts',(-1.10595102243643,-0.0762225747374254,
0.199591971170104));
#24382=CARTESIAN_POINT('Ctrl Pts',(-1.10653577764992,-0.0595300000000001,
0.196295654879792));
#24383=CARTESIAN_POINT('',(-1.123812,-0.05953,1.37627276864339E-16));
#24384=CARTESIAN_POINT('Origin',(0.,-0.05953,0.));
#24385=CARTESIAN_POINT('',(-1.123812,-0.35718,1.37627276864339E-16));
#24386=CARTESIAN_POINT('',(-1.123812,-0.208355,1.37627276864339E-16));
#24387=CARTESIAN_POINT('Origin',(0.,-0.35718,0.));
#24388=CARTESIAN_POINT('',(-1.10653577764992,-0.05953,-0.196295654879793));
#24389=CARTESIAN_POINT('Origin',(0.,-0.05953,0.));
#24390=CARTESIAN_POINT('',(-0.843383895613249,-0.05953,-0.742736168477219));
#24391=CARTESIAN_POINT('Ctrl Pts',(-1.10653577764992,-0.0595300000000001,
-0.196295654879792));
#24392=CARTESIAN_POINT('Ctrl Pts',(-1.10595102243643,-0.0762225747374255,
-0.199591971170104));
#24393=CARTESIAN_POINT('Ctrl Pts',(-1.10509821673782,-0.0928409665394228,
-0.204327142733962));
#24394=CARTESIAN_POINT('Ctrl Pts',(-1.10139388218929,-0.144299303100741,
-0.22376314604679));
#24395=CARTESIAN_POINT('Ctrl Pts',(-1.09728268713976,-0.177024326825049,
-0.243890930799338));
#24396=CARTESIAN_POINT('Ctrl Pts',(-1.08664560412098,-0.227269801620063,
-0.287406530683753));
#24397=CARTESIAN_POINT('Ctrl Pts',(-1.0788165083757,-0.251265615809407,
-0.316022600643821));
#24398=CARTESIAN_POINT('Ctrl Pts',(-1.06356957703048,-0.279889827963178,
-0.363699428370918));
#24399=CARTESIAN_POINT('Ctrl Pts',(-1.05494634094458,-0.290879136862659,
-0.388295406390235));
#24400=CARTESIAN_POINT('Ctrl Pts',(-1.03504317708586,-0.305251990234488,
-0.438600874831839));
#24401=CARTESIAN_POINT('Ctrl Pts',(-1.02374168767024,-0.308638795020976,
-0.46430090015576));
#24402=CARTESIAN_POINT('Ctrl Pts',(-1.00129756308006,-0.308638795020976,
-0.510906605094603));
#24403=CARTESIAN_POINT('Ctrl Pts',(-0.988250837578047,-0.305251990234488,
-0.535766169015486));
#24404=CARTESIAN_POINT('Ctrl Pts',(-0.961329858300736,-0.290879136862659,
-0.582692035672022));
#24405=CARTESIAN_POINT('Ctrl Pts',(-0.947476448101718,-0.279889827963178,
-0.604769294586516));
#24406=CARTESIAN_POINT('Ctrl Pts',(-0.919707509403859,-0.251265615809407,
-0.646415841396062));
#24407=CARTESIAN_POINT('Ctrl Pts',(-0.902215926359523,-0.227269801620064,
-0.670378702718353));
#24408=CARTESIAN_POINT('Ctrl Pts',(-0.87482617317514,-0.177024326825049,
-0.705826641853758));
#24409=CARTESIAN_POINT('Ctrl Pts',(-0.861652925570091,-0.144299303100741,
-0.721590372101268));
#24410=CARTESIAN_POINT('Ctrl Pts',(-0.848766861100456,-0.0928409665394229,
-0.736604687327351));
#24411=CARTESIAN_POINT('Ctrl Pts',(-0.84559647055299,-0.0762225747374255,
-0.740223768851063));
#24412=CARTESIAN_POINT('Ctrl Pts',(-0.843383895613249,-0.0595300000000001,
-0.742736168477219));
#24413=CARTESIAN_POINT('',(-0.536443649899847,-0.05953,-0.987512846410683));
#24414=CARTESIAN_POINT('Origin',(0.,-0.05953,0.));
#24415=CARTESIAN_POINT('',(0.0548532617164172,-0.05953,-1.12247250791415));
#24416=CARTESIAN_POINT('Ctrl Pts',(-0.536443649899848,-0.0595300000000001,
-0.987512846410683));
#24417=CARTESIAN_POINT('Ctrl Pts',(-0.533501897135712,-0.0762225747374254,
-0.989110885965947));
#24418=CARTESIAN_POINT('Ctrl Pts',(-0.529268075276156,-0.0928409665394227,
-0.991396466802469));
#24419=CARTESIAN_POINT('Ctrl Pts',(-0.511762781179147,-0.144299303100741,
-1.00061845128527));
#24420=CARTESIAN_POINT('Ctrl Pts',(-0.493462957200432,-0.177024326825049,
-1.0099536580922));
#24421=CARTESIAN_POINT('Ctrl Pts',(-0.45280897844858,-0.227269801620063,
-1.02876878445619));
#24422=CARTESIAN_POINT('Ctrl Pts',(-0.425554672694337,-0.251265615809407,
-1.04048957871266));
#24423=CARTESIAN_POINT('Ctrl Pts',(-0.3787731215897,-0.279889827963178,
-1.05829506364875));
#24424=CARTESIAN_POINT('Ctrl Pts',(-0.354166711873529,-0.290879136862659,
-1.06688848765783));
#24425=CARTESIAN_POINT('Ctrl Pts',(-0.302426893214944,-0.305251990234488,
-1.08269251410343));
#24426=CARTESIAN_POINT('Ctrl Pts',(-0.275287440920027,-0.308638795020976,
-1.0898803575765));
#24427=CARTESIAN_POINT('Ctrl Pts',(-0.224855950742601,-0.308638795020976,
-1.10139101611326));
#24428=CARTESIAN_POINT('Ctrl Pts',(-0.19728546073067,-0.305251990234488,
-1.10669035995599));
#24429=CARTESIAN_POINT('Ctrl Pts',(-0.143812384801039,-0.290879136862659,
-1.11490049012186));
#24430=CARTESIAN_POINT('Ctrl Pts',(-0.117914228755037,-0.279889827963178,
-1.1178344036749));
#24431=CARTESIAN_POINT('Ctrl Pts',(-0.0680399972366989,-0.251265615809407,
-1.12208997038458));
#24432=CARTESIAN_POINT('Ctrl Pts',(-0.0383992541984084,-0.227269801620063,
-1.12335509974011));
#24433=CARTESIAN_POINT('Ctrl Pts',(0.00639229239215326,-0.177024326825049,
-1.12404235695137));
#24434=CARTESIAN_POINT('Ctrl Pts',(0.0269302585198977,-0.144299303100741,
-1.12357162229597));
#24435=CARTESIAN_POINT('Ctrl Pts',(0.04670325263426,-0.0928409665394228,
-1.12285816383385));
#24436=CARTESIAN_POINT('Ctrl Pts',(0.0515094706813703,-0.0762225747374255,
-1.12263591311425));
#24437=CARTESIAN_POINT('Ctrl Pts',(0.0548532617164176,-0.0595300000000001,
-1.12247250791414));
#24438=CARTESIAN_POINT('',(0.437601487681057,-0.05953,-1.03511272300331));
#24439=CARTESIAN_POINT('Origin',(0.,-0.05953,0.));
#24440=CARTESIAN_POINT('',(0.911784794170997,-0.05953,-0.656964154625313));
#24441=CARTESIAN_POINT('Ctrl Pts',(0.437601487681056,-0.0595300000000001,
-1.03511272300331));
#24442=CARTESIAN_POINT('Ctrl Pts',(0.440685038163619,-0.0762225747374255,
-1.03380912944435));
#24443=CARTESIAN_POINT('Ctrl Pts',(0.445111721969657,-0.0928409665394228,
-1.03192403056628));
#24444=CARTESIAN_POINT('Ctrl Pts',(0.463236132117164,-0.144299303100741,
-1.0239876538093));
#24445=CARTESIAN_POINT('Ctrl Pts',(0.481944444320713,-0.177024326825049,
-1.01550068154148));
#24446=CARTESIAN_POINT('Ctrl Pts',(0.522002043615455,-0.227269801620064,
-0.995447160474328));
#24447=CARTESIAN_POINT('Ctrl Pts',(0.548158511259203,-0.251265615809407,
-0.981446681891443));
#24448=CARTESIAN_POINT('Ctrl Pts',(0.591247219971725,-0.279889827963178,
-0.955972930713954));
#24449=CARTESIAN_POINT('Ctrl Pts',(0.613307674922609,-0.290879136862659,
-0.942092777160053));
#24450=CARTESIAN_POINT('Ctrl Pts',(0.657923009631182,-0.305251990234487,
-0.91149460735272));
#24451=CARTESIAN_POINT('Ctrl Pts',(0.680463863683393,-0.308638795020976,
-0.894757676234429));
#24452=CARTESIAN_POINT('Ctrl Pts',(0.720906778729542,-0.308638795020976,
-0.862505527716294));
#24453=CARTESIAN_POINT('Ctrl Pts',(0.742239891936899,-0.305251990234488,
-0.844254137480381));
#24454=CARTESIAN_POINT('Ctrl Pts',(0.781998747691872,-0.290879136862659,
-0.80756613568454));
#24455=CARTESIAN_POINT('Ctrl Pts',(0.800439809856112,-0.279889827963178,
-0.789147407129765));
#24456=CARTESIAN_POINT('Ctrl Pts',(0.834863020612702,-0.251265615809407,
-0.752807465209441));
#24457=CARTESIAN_POINT('Ctrl Pts',(0.854332839576145,-0.227269801620064,
-0.73042219438957));
#24458=CARTESIAN_POINT('Ctrl Pts',(0.882797231409153,-0.177024326825049,
-0.695831250979106));
#24459=CARTESIAN_POINT('Ctrl Pts',(0.895234408667242,-0.144299303100741,
-0.679480524217551));
#24460=CARTESIAN_POINT('Ctrl Pts',(0.907004864562642,-0.0928409665394228,
-0.663576540841106));
#24461=CARTESIAN_POINT('Ctrl Pts',(0.909827729890942,-0.0762225747374256,
-0.659680317203144));
#24462=CARTESIAN_POINT('Ctrl Pts',(0.911784794170998,-0.0595300000000001,
-0.656964154625312));
#24463=CARTESIAN_POINT('',(1.08212377959455,-0.05953,-0.303251606722892));
#24464=CARTESIAN_POINT('Origin',(0.,-0.05953,0.));
#24465=CARTESIAN_POINT('',(1.08212377959455,-0.05953,0.303251606722892));
#24466=CARTESIAN_POINT('Ctrl Pts',(1.08212377959455,-0.0595300000000001,
-0.303251606722892));
#24467=CARTESIAN_POINT('Ctrl Pts',(1.0830271513892,-0.0762225747374255,
-0.300028012588062));
#24468=CARTESIAN_POINT('Ctrl Pts',(1.08431331394788,-0.0928409665394228,
-0.2953917518996));
#24469=CARTESIAN_POINT('Ctrl Pts',(1.08940878963422,-0.144299303100741,
-0.276273267473431));
#24470=CARTESIAN_POINT('Ctrl Pts',(1.09443784939331,-0.177024326825049,
-0.256354979351213));
#24471=CARTESIAN_POINT('Ctrl Pts',(1.10373487993589,-0.227269801620064,
-0.212533521233765));
#24472=CARTESIAN_POINT('Ctrl Pts',(1.10909715583869,-0.251265615809407,
-0.183354415742157));
#24473=CARTESIAN_POINT('Ctrl Pts',(1.1160463456491,-0.279889827963178,-0.133783682657561));
#24474=CARTESIAN_POINT('Ctrl Pts',(1.11894887330541,-0.290879136862659,
-0.107881990270302));
#24475=CARTESIAN_POINT('Ctrl Pts',(1.12284346704144,-0.305251990234488,
-0.0539226701638766));
#24476=CARTESIAN_POINT('Ctrl Pts',(1.123812,-0.308638795020976,-0.025864214957475));
#24477=CARTESIAN_POINT('Ctrl Pts',(1.123812,-0.308638795020976,0.025864214957475));
#24478=CARTESIAN_POINT('Ctrl Pts',(1.12284346704144,-0.305251990234488,
0.0539226701638766));
#24479=CARTESIAN_POINT('Ctrl Pts',(1.11894887330541,-0.290879136862659,
0.107881990270302));
#24480=CARTESIAN_POINT('Ctrl Pts',(1.1160463456491,-0.279889827963178,0.133783682657561));
#24481=CARTESIAN_POINT('Ctrl Pts',(1.10909715583869,-0.251265615809407,
0.183354415742157));
#24482=CARTESIAN_POINT('Ctrl Pts',(1.10373487993589,-0.227269801620064,
0.212533521233765));
#24483=CARTESIAN_POINT('Ctrl Pts',(1.09443784939331,-0.177024326825049,
0.256354979351213));
#24484=CARTESIAN_POINT('Ctrl Pts',(1.08940878963422,-0.144299303100741,
0.276273267473431));
#24485=CARTESIAN_POINT('Ctrl Pts',(1.08431331394788,-0.0928409665394228,
0.2953917518996));
#24486=CARTESIAN_POINT('Ctrl Pts',(1.0830271513892,-0.0762225747374255,
0.300028012588062));
#24487=CARTESIAN_POINT('Ctrl Pts',(1.08212377959455,-0.0595300000000001,
0.303251606722892));
#24488=CARTESIAN_POINT('Origin',(0.,-0.05953,0.));
#24489=CARTESIAN_POINT('Origin',(0.,-0.05953,0.));
#24490=CARTESIAN_POINT('',(0.0589974094846122,-0.05953,1.07456964270265));
#24491=CARTESIAN_POINT('Origin',(0.,-0.05953,0.));
#24492=CARTESIAN_POINT('Origin',(-0.244773027351946,-0.05953,1.07242070340001));
#24493=CARTESIAN_POINT('Origin',(-0.244773027351946,0.,1.07242070340001));
#24494=CARTESIAN_POINT('',(-0.519393123750572,-0.05953,0.942555777842682));
#24495=CARTESIAN_POINT('Ctrl Pts',(-0.519393123750572,-0.05953,0.942555777842682));
#24496=CARTESIAN_POINT('Ctrl Pts',(-0.513714466572041,-0.0925528133349865,
0.945684988399766));
#24497=CARTESIAN_POINT('Ctrl Pts',(-0.503136848051455,-0.124911173756694,
0.951483858396181));
#24498=CARTESIAN_POINT('Ctrl Pts',(-0.47593627990192,-0.177924977804098,
0.965323333309091));
#24499=CARTESIAN_POINT('Ctrl Pts',(-0.460931856495794,-0.199697230012983,
0.972669835243841));
#24500=CARTESIAN_POINT('Ctrl Pts',(-0.426157505475872,-0.237895043532788,
0.988400002689705));
#24501=CARTESIAN_POINT('Ctrl Pts',(-0.406380688682952,-0.254319232363049,
0.996771768218699));
#24502=CARTESIAN_POINT('Ctrl Pts',(-0.364750145543744,-0.28018331644634,
1.01272583306292));
#24503=CARTESIAN_POINT('Ctrl Pts',(-0.340838910881557,-0.29104845371857,
1.02112815447116));
#24504=CARTESIAN_POINT('Ctrl Pts',(-0.290495481564827,-0.30527573347708,
1.036574285215));
#24505=CARTESIAN_POINT('Ctrl Pts',(-0.264056468041074,-0.308638795020976,
1.04359501395068));
#24506=CARTESIAN_POINT('Ctrl Pts',(-0.214892249704082,-0.308638795020976,
1.05481642595959));
#24507=CARTESIAN_POINT('Ctrl Pts',(-0.188025341585962,-0.30527573347708,
1.05996242598502));
#24508=CARTESIAN_POINT('Ctrl Pts',(-0.135965654106109,-0.29104845371857,
1.06788913840721));
#24509=CARTESIAN_POINT('Ctrl Pts',(-0.110776745452494,-0.28018331644634,
1.07069360430242));
#24510=CARTESIAN_POINT('Ctrl Pts',(-0.0663467128214646,-0.254319232363049,
1.07438230428002));
#24511=CARTESIAN_POINT('Ctrl Pts',(-0.0448960436540983,-0.237895043532788,
1.07542044338697));
#24512=CARTESIAN_POINT('Ctrl Pts',(-0.00674037211528124,-0.199697230012983,
1.07633607767727));
#24513=CARTESIAN_POINT('Ctrl Pts',(0.00996567398334777,-0.177924977804098,
1.07622728347683));
#24514=CARTESIAN_POINT('Ctrl Pts',(0.0404772621979741,-0.124911173756694,
1.07556023164702));
#24515=CARTESIAN_POINT('Ctrl Pts',(0.0525234025782719,-0.0925528133349865,
1.07492508698591));
#24516=CARTESIAN_POINT('Ctrl Pts',(0.0589974094846124,-0.05953,1.07456964270265));
#24517=CARTESIAN_POINT('Origin',(-0.244773027351946,-0.05953,1.07242070340001));
#24518=CARTESIAN_POINT('Origin',(0.,-0.05953,0.));
#24519=CARTESIAN_POINT('',(-0.803348093619616,-0.05953,0.716109245731214));
#24520=CARTESIAN_POINT('Origin',(0.,-0.05953,0.));
#24521=CARTESIAN_POINT('Origin',(-0.991065754692661,-0.05953,0.477272113029314));
#24522=CARTESIAN_POINT('Origin',(-0.991065754692661,0.,0.477272113029314));
#24523=CARTESIAN_POINT('',(-1.06075609691358,-0.05953,0.181596019242328));
#24524=CARTESIAN_POINT('Ctrl Pts',(-1.06075609691358,-0.05953,0.181596019242328));
#24525=CARTESIAN_POINT('Ctrl Pts',(-1.05966202740332,-0.0925528133349865,
0.187986803072856));
#24526=CARTESIAN_POINT('Ctrl Pts',(-1.05760072925372,-0.124911173756694,
0.199872254546857));
#24527=CARTESIAN_POINT('Ctrl Pts',(-1.05146158959546,-0.177924977804098,
0.22976728653846));
#24528=CARTESIAN_POINT('Ctrl Pts',(-1.04785021111757,-0.199697230012983,
0.246078686169301));
#24529=CARTESIAN_POINT('Ctrl Pts',(-1.03846709802406,-0.237895043532788,
0.283073967563097));
#24530=CARTESIAN_POINT('Ctrl Pts',(-1.03268176429485,-0.254319232363049,
0.303755815985685));
#24531=CARTESIAN_POINT('Ctrl Pts',(-1.01919893537026,-0.28018331644634,
0.346251081972725));
#24532=CARTESIAN_POINT('Ctrl Pts',(-1.01085972381132,-0.29104845371857,
0.370184399726282));
#24533=CARTESIAN_POINT('Ctrl Pts',(-0.99154738033959,-0.30527573347708,
0.419174982698463));
#24534=CARTESIAN_POINT('Ctrl Pts',(-0.980551951791748,-0.308638795020976,
0.444223188605045));
#24535=CARTESIAN_POINT('Ctrl Pts',(-0.958671816228589,-0.308638795020976,
0.489657758261848));
#24536=CARTESIAN_POINT('Ctrl Pts',(-0.945943877838127,-0.30527573347708,
0.51387163140139));
#24537=CARTESIAN_POINT('Ctrl Pts',(-0.91968254693063,-0.29104845371857,
0.559515758398093));
#24538=CARTESIAN_POINT('Ctrl Pts',(-0.906170138993533,-0.28018331644634,
0.580957796077825));
#24539=CARTESIAN_POINT('Ctrl Pts',(-0.8813524085237,-0.254319232363049,
0.617994461173994));
#24540=CARTESIAN_POINT('Ctrl Pts',(-0.868789784891799,-0.237895043532788,
0.635412538795143));
#24541=CARTESIAN_POINT('Ctrl Pts',(-0.845715984518854,-0.199697230012983,
0.66581473268113));
#24542=CARTESIAN_POINT('Ctrl Pts',(-0.835214876415962,-0.177924977804098,
0.678808213394124));
#24543=CARTESIAN_POINT('Ctrl Pts',(-0.815669690204649,-0.124911173756694,
0.702247233627224));
#24544=CARTESIAN_POINT('Ctrl Pts',(-0.807662468433796,-0.0925528133349865,
0.711269279199861));
#24545=CARTESIAN_POINT('Ctrl Pts',(-0.803348093619616,-0.05953,0.716109245731214));
#24546=CARTESIAN_POINT('Origin',(-0.991065754692661,-0.05953,0.477272113029314));
#24547=CARTESIAN_POINT('Origin',(0.,-0.05953,0.));
#24548=CARTESIAN_POINT('',(-1.076188,-0.05953,1.31795018948079E-16));
#24549=CARTESIAN_POINT('Origin',(0.,-0.05953,0.));
#24550=CARTESIAN_POINT('',(-1.06075609691358,-0.05953,-0.181596019242328));
#24551=CARTESIAN_POINT('Origin',(0.,-0.05953,0.));
#24552=CARTESIAN_POINT('Origin',(-0.991065754692661,-0.05953,-0.477272113029314));
#24553=CARTESIAN_POINT('Origin',(-0.991065754692661,0.,-0.477272113029314));
#24554=CARTESIAN_POINT('',(-0.803348093619616,-0.05953,-0.716109245731215));
#24555=CARTESIAN_POINT('Ctrl Pts',(-0.803348093619616,-0.05953,-0.716109245731215));
#24556=CARTESIAN_POINT('Ctrl Pts',(-0.807662468433795,-0.0925528133349865,
-0.711269279199862));
#24557=CARTESIAN_POINT('Ctrl Pts',(-0.815669690204649,-0.124911173756694,
-0.702247233627224));
#24558=CARTESIAN_POINT('Ctrl Pts',(-0.835214876415962,-0.177924977804098,
-0.678808213394124));
#24559=CARTESIAN_POINT('Ctrl Pts',(-0.845715984518854,-0.199697230012983,
-0.66581473268113));
#24560=CARTESIAN_POINT('Ctrl Pts',(-0.868789784891799,-0.237895043532788,
-0.635412538795143));
#24561=CARTESIAN_POINT('Ctrl Pts',(-0.8813524085237,-0.254319232363049,
-0.617994461173994));
#24562=CARTESIAN_POINT('Ctrl Pts',(-0.906170138993533,-0.28018331644634,
-0.580957796077826));
#24563=CARTESIAN_POINT('Ctrl Pts',(-0.91968254693063,-0.29104845371857,
-0.559515758398093));
#24564=CARTESIAN_POINT('Ctrl Pts',(-0.945943877838127,-0.30527573347708,
-0.51387163140139));
#24565=CARTESIAN_POINT('Ctrl Pts',(-0.958671816228589,-0.308638795020976,
-0.489657758261848));
#24566=CARTESIAN_POINT('Ctrl Pts',(-0.980551951791748,-0.308638795020976,
-0.444223188605045));
#24567=CARTESIAN_POINT('Ctrl Pts',(-0.99154738033959,-0.30527573347708,
-0.419174982698463));
#24568=CARTESIAN_POINT('Ctrl Pts',(-1.01085972381132,-0.29104845371857,
-0.370184399726282));
#24569=CARTESIAN_POINT('Ctrl Pts',(-1.01919893537026,-0.28018331644634,
-0.346251081972725));
#24570=CARTESIAN_POINT('Ctrl Pts',(-1.03268176429485,-0.254319232363049,
-0.303755815985685));
#24571=CARTESIAN_POINT('Ctrl Pts',(-1.03846709802406,-0.237895043532788,
-0.283073967563097));
#24572=CARTESIAN_POINT('Ctrl Pts',(-1.04785021111757,-0.199697230012983,
-0.246078686169302));
#24573=CARTESIAN_POINT('Ctrl Pts',(-1.05146158959546,-0.177924977804098,
-0.229767286538461));
#24574=CARTESIAN_POINT('Ctrl Pts',(-1.05760072925372,-0.124911173756694,
-0.199872254546858));
#24575=CARTESIAN_POINT('Ctrl Pts',(-1.05966202740332,-0.0925528133349864,
-0.187986803072857));
#24576=CARTESIAN_POINT('Ctrl Pts',(-1.06075609691358,-0.05953,-0.181596019242328));
#24577=CARTESIAN_POINT('Origin',(-0.991065754692661,-0.05953,-0.477272113029314));
#24578=CARTESIAN_POINT('Origin',(0.,-0.05953,0.));
#24579=CARTESIAN_POINT('',(-0.519393123750572,-0.05953,-0.942555777842682));
#24580=CARTESIAN_POINT('Origin',(0.,-0.05953,0.));
#24581=CARTESIAN_POINT('Origin',(-0.244773027351946,-0.05953,-1.07242070340001));
#24582=CARTESIAN_POINT('Origin',(-0.244773027351946,0.,-1.07242070340001));
#24583=CARTESIAN_POINT('',(0.0589974094846125,-0.05953,-1.07456964270265));
#24584=CARTESIAN_POINT('Ctrl Pts',(0.0589974094846127,-0.05953,-1.07456964270265));
#24585=CARTESIAN_POINT('Ctrl Pts',(0.0525234025782722,-0.0925528133349865,
-1.07492508698591));
#24586=CARTESIAN_POINT('Ctrl Pts',(0.0404772621979744,-0.124911173756694,
-1.07556023164702));
#24587=CARTESIAN_POINT('Ctrl Pts',(0.0099656739833481,-0.177924977804098,
-1.07622728347683));
#24588=CARTESIAN_POINT('Ctrl Pts',(-0.00674037211528096,-0.199697230012983,
-1.07633607767727));
#24589=CARTESIAN_POINT('Ctrl Pts',(-0.044896043654098,-0.237895043532788,
-1.07542044338697));
#24590=CARTESIAN_POINT('Ctrl Pts',(-0.0663467128214644,-0.254319232363049,
-1.07438230428002));
#24591=CARTESIAN_POINT('Ctrl Pts',(-0.110776745452493,-0.28018331644634,
-1.07069360430242));
#24592=CARTESIAN_POINT('Ctrl Pts',(-0.135965654106109,-0.29104845371857,
-1.06788913840721));
#24593=CARTESIAN_POINT('Ctrl Pts',(-0.188025341585962,-0.30527573347708,
-1.05996242598502));
#24594=CARTESIAN_POINT('Ctrl Pts',(-0.214892249704082,-0.308638795020976,
-1.05481642595959));
#24595=CARTESIAN_POINT('Ctrl Pts',(-0.264056468041074,-0.308638795020976,
-1.04359501395068));
#24596=CARTESIAN_POINT('Ctrl Pts',(-0.290495481564827,-0.30527573347708,
-1.036574285215));
#24597=CARTESIAN_POINT('Ctrl Pts',(-0.340838910881557,-0.291048453718569,
-1.02112815447116));
#24598=CARTESIAN_POINT('Ctrl Pts',(-0.364750145543744,-0.28018331644634,
-1.01272583306292));
#24599=CARTESIAN_POINT('Ctrl Pts',(-0.406380688682952,-0.254319232363049,
-0.996771768218699));
#24600=CARTESIAN_POINT('Ctrl Pts',(-0.426157505475872,-0.237895043532788,
-0.988400002689705));
#24601=CARTESIAN_POINT('Ctrl Pts',(-0.460931856495794,-0.199697230012983,
-0.972669835243841));
#24602=CARTESIAN_POINT('Ctrl Pts',(-0.475936279901919,-0.177924977804098,
-0.965323333309091));
#24603=CARTESIAN_POINT('Ctrl Pts',(-0.503136848051454,-0.124911173756694,
-0.951483858396181));
#24604=CARTESIAN_POINT('Ctrl Pts',(-0.513714466572041,-0.0925528133349865,
-0.945684988399766));
#24605=CARTESIAN_POINT('Ctrl Pts',(-0.519393123750572,-0.05953,-0.942555777842682));
#24606=CARTESIAN_POINT('Origin',(-0.244773027351946,-0.05953,-1.07242070340001));
#24607=CARTESIAN_POINT('Origin',(0.,-0.05953,0.));
#24608=CARTESIAN_POINT('',(0.413083465285518,-0.05953,-0.993751811093549));
#24609=CARTESIAN_POINT('Origin',(0.,-0.05953,0.));
#24610=CARTESIAN_POINT('Origin',(0.685838782044607,-0.05953,-0.860014630714833));
#24611=CARTESIAN_POINT('Origin',(0.685838782044607,0.,-0.860014630714833));
#24612=CARTESIAN_POINT('',(0.876916659919095,-0.05953,-0.623857181492959));
#24613=CARTESIAN_POINT('Ctrl Pts',(0.876916659919095,-0.05953,-0.623857181492958));
#24614=CARTESIAN_POINT('Ctrl Pts',(0.873158080166742,-0.0925528133349865,
-0.62914037979579));
#24615=CARTESIAN_POINT('Ctrl Pts',(0.866144010579847,-0.124911173756694,
-0.638954437806245));
#24616=CARTESIAN_POINT('Ctrl Pts',(0.847641868610495,-0.177924977804098,
-0.663225258065736));
#24617=CARTESIAN_POINT('Ctrl Pts',(0.837310877969633,-0.199697230012983,
-0.676354402927683));
#24618=CARTESIAN_POINT('Ctrl Pts',(0.81280533416753,-0.237895043532788,
-0.705614819529209));
#24619=CARTESIAN_POINT('Ctrl Pts',(0.798619410861634,-0.254319232363049,
-0.721738358858166));
#24620=CARTESIAN_POINT('Ctrl Pts',(0.768033796848072,-0.28018331644634,
-0.754175290318038));
#24621=CARTESIAN_POINT('Ctrl Pts',(0.750136149454208,-0.29104845371857,
-0.772120216227122));
#24622=CARTESIAN_POINT('Ctrl Pts',(0.711480111898423,-0.30527573347708,
-0.807879894508811));
#24623=CARTESIAN_POINT('Ctrl Pts',(0.690705563850638,-0.308638795020976,
-0.825676810575913));
#24624=CARTESIAN_POINT('Ctrl Pts',(0.651278921914856,-0.308638795020976,
-0.857118508332695));
#24625=CARTESIAN_POINT('Ctrl Pts',(0.629305439856167,-0.30527573347708,
-0.873412008702649));
#24626=CARTESIAN_POINT('Ctrl Pts',(0.585840553788742,-0.29104845371857,
-0.903141581680914));
#24627=CARTESIAN_POINT('Ctrl Pts',(0.564362943424239,-0.28018331644634,
-0.916597376014514));
#24628=CARTESIAN_POINT('Ctrl Pts',(0.525933334162556,-0.254319232363049,
-0.939198248544427));
#24629=CARTESIAN_POINT('Ctrl Pts',(0.507057380724533,-0.237895043532788,
-0.949440676105255));
#24630=CARTESIAN_POINT('Ctrl Pts',(0.473077587363686,-0.199697230012983,
-0.966820759530997));
#24631=CARTESIAN_POINT('Ctrl Pts',(0.457978755888596,-0.177924977804098,
-0.973971221090534));
#24632=CARTESIAN_POINT('Ctrl Pts',(0.430199341854858,-0.124911173756694,
-0.986608710139579));
#24633=CARTESIAN_POINT('Ctrl Pts',(0.419070565453384,-0.0925528133349865,
-0.991263089003441));
#24634=CARTESIAN_POINT('Ctrl Pts',(0.413083465285518,-0.05953,-0.993751811093549));
#24635=CARTESIAN_POINT('Origin',(0.685838782044607,-0.05953,-0.860014630714833));
#24636=CARTESIAN_POINT('Origin',(0.,-0.208355,0.));
#24637=CARTESIAN_POINT('',(-1.076188,-0.35718,1.31795018948079E-16));
#24638=CARTESIAN_POINT('Origin',(0.,-0.35718,0.));
#24639=CARTESIAN_POINT('',(-1.076188,-0.208355,1.31795018948079E-16));
#24640=CARTESIAN_POINT('',(1.03449977959455,-0.05953,0.296632461748266));
#24641=CARTESIAN_POINT('Origin',(0.,-0.05953,0.));
#24642=CARTESIAN_POINT('',(1.03449977959455,-0.05953,-0.296632461748266));
#24643=CARTESIAN_POINT('Ctrl Pts',(1.03449977959455,-0.05953,0.296632461748267));
#24644=CARTESIAN_POINT('Ctrl Pts',(1.03628691421076,-0.0925528133349865,
0.290399865505497));
#24645=CARTESIAN_POINT('Ctrl Pts',(1.03958665287714,-0.124911173756694,
0.278797079997872));
#24646=CARTESIAN_POINT('Ctrl Pts',(1.0470264474309,-0.177924977804098,0.249198913998601));
#24647=CARTESIAN_POINT('Ctrl Pts',(1.05084995891418,-0.199697230012983,
0.232935932341942));
#24648=CARTESIAN_POINT('Ctrl Pts',(1.05844771715377,-0.237895043532788,
0.195533155353269));
#24649=CARTESIAN_POINT('Ctrl Pts',(1.06220882929878,-0.254319232363049,
0.17438929156337));
#24650=CARTESIAN_POINT('Ctrl Pts',(1.06849922508772,-0.28018331644634,0.130252399648131));
#24651=CARTESIAN_POINT('Ctrl Pts',(1.07137013248666,-0.29104845371857,0.105070977154072));
#24652=CARTESIAN_POINT('Ctrl Pts',(1.07522652957392,-0.30527573347708,0.0525526752791107));
#24653=CARTESIAN_POINT('Ctrl Pts',(1.076188,-0.308638795020976,0.025214283908933));
#24654=CARTESIAN_POINT('Ctrl Pts',(1.076188,-0.308638795020976,-0.025214283908933));
#24655=CARTESIAN_POINT('Ctrl Pts',(1.07522652957392,-0.30527573347708,-0.0525526752791107));
#24656=CARTESIAN_POINT('Ctrl Pts',(1.07137013248666,-0.29104845371857,-0.105070977154072));
#24657=CARTESIAN_POINT('Ctrl Pts',(1.06849922508772,-0.28018331644634,-0.130252399648131));
#24658=CARTESIAN_POINT('Ctrl Pts',(1.06220882929878,-0.254319232363049,
-0.17438929156337));
#24659=CARTESIAN_POINT('Ctrl Pts',(1.05844771715377,-0.237895043532788,
-0.195533155353269));
#24660=CARTESIAN_POINT('Ctrl Pts',(1.05084995891418,-0.199697230012983,
-0.232935932341942));
#24661=CARTESIAN_POINT('Ctrl Pts',(1.0470264474309,-0.177924977804098,-0.249198913998601));
#24662=CARTESIAN_POINT('Ctrl Pts',(1.03958665287714,-0.124911173756694,
-0.278797079997872));
#24663=CARTESIAN_POINT('Ctrl Pts',(1.03628691421076,-0.0925528133349865,
-0.290399865505497));
#24664=CARTESIAN_POINT('Ctrl Pts',(1.03449977959455,-0.05953,-0.296632461748267));
#24665=CARTESIAN_POINT('Origin',(0.,-0.05953,0.));
#24666=CARTESIAN_POINT('Origin',(0.,-0.05953,0.));
#24667=CARTESIAN_POINT('Origin',(1.1,-0.05953,0.));
#24668=CARTESIAN_POINT('Origin',(1.1,0.,0.));
#24669=CARTESIAN_POINT('Origin',(1.1,-0.05953,0.));
#24670=CARTESIAN_POINT('Origin',(0.,-0.35718,0.));
#24671=CARTESIAN_POINT('Origin',(0.,-0.05953,0.));
#73262=UNCERTAINTY_MEASURE_WITH_UNIT(LENGTH_MEASURE(0.001),#73367,
'DISTANCE_ACCURACY_VALUE',
'Maximum model space distance between geometric entities at asserted c
onnectivities');
#73302=UNCERTAINTY_MEASURE_WITH_UNIT(LENGTH_MEASURE(0.001),#73367,
'DISTANCE_ACCURACY_VALUE',
'Maximum model space distance between geometric entities at asserted c
onnectivities');
#73326=(
GEOMETRIC_REPRESENTATION_CONTEXT(3)
GLOBAL_UNCERTAINTY_ASSIGNED_CONTEXT((#73262))
GLOBAL_UNIT_ASSIGNED_CONTEXT((#73367,#73369,#73370))
REPRESENTATION_CONTEXT('','3D')
);
#73366=(
GEOMETRIC_REPRESENTATION_CONTEXT(3)
GLOBAL_UNCERTAINTY_ASSIGNED_CONTEXT((#73302))
GLOBAL_UNIT_ASSIGNED_CONTEXT((#73367,#73369,#73370))
REPRESENTATION_CONTEXT('','3D')
);
#73367=(
LENGTH_UNIT()
NAMED_UNIT(*)
SI_UNIT(.CENTI.,.METRE.)
);
#73369=(
NAMED_UNIT(*)
PLANE_ANGLE_UNIT()
SI_UNIT($,.RADIAN.)
);
#73370=(
NAMED_UNIT(*)
SI_UNIT($,.STERADIAN.)
SOLID_ANGLE_UNIT()
);
#73394=SHAPE_DEFINITION_REPRESENTATION(#73457,#73630);
#73457=PRODUCT_DEFINITION_SHAPE('',$,#73694);
#73630=SHAPE_REPRESENTATION('',(#17472),#73326);
#73670=PRODUCT_DEFINITION_CONTEXT('part definition',#73861,'design');
#73694=PRODUCT_DEFINITION('Cage','Cage',#73757,#73670);
#73757=PRODUCT_DEFINITION_FORMATION('',$,#73886);
#73861=APPLICATION_CONTEXT(
'Core Data for Automotive Mechanical Design Process');
#73862=PRODUCT_CONTEXT('part definition',#73861,'mechanical');
#73886=PRODUCT('Cage','Cage','Cage',(#73862));
#73982=COLOUR_RGB('Grey',0.48,0.52,0.57);
#73983=FILL_AREA_STYLE_COLOUR('',#73982);
#73984=FILL_AREA_STYLE('',(#73983));
#73985=SURFACE_STYLE_FILL_AREA(#73984);
#73986=SURFACE_SIDE_STYLE('',(#73985));
#73987=SURFACE_STYLE_USAGE(.BOTH.,#73986);
#73988=PRESENTATION_STYLE_ASSIGNMENT((#73987));
ENDSEC;
END-ISO-10303-21;
